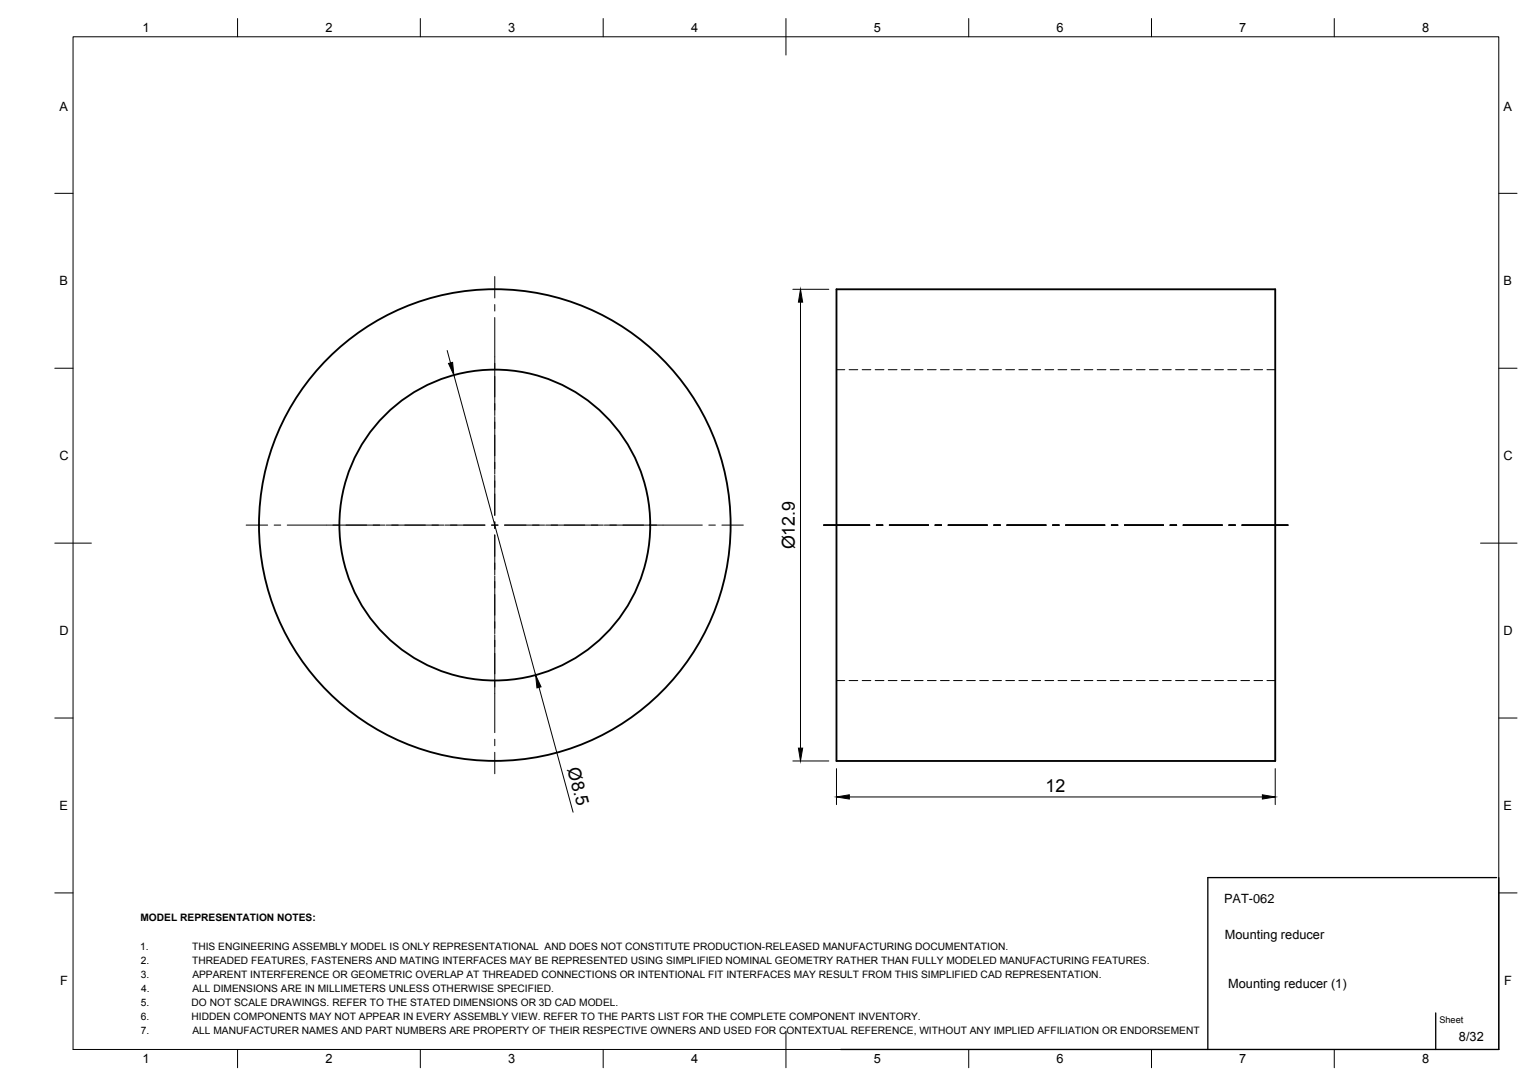
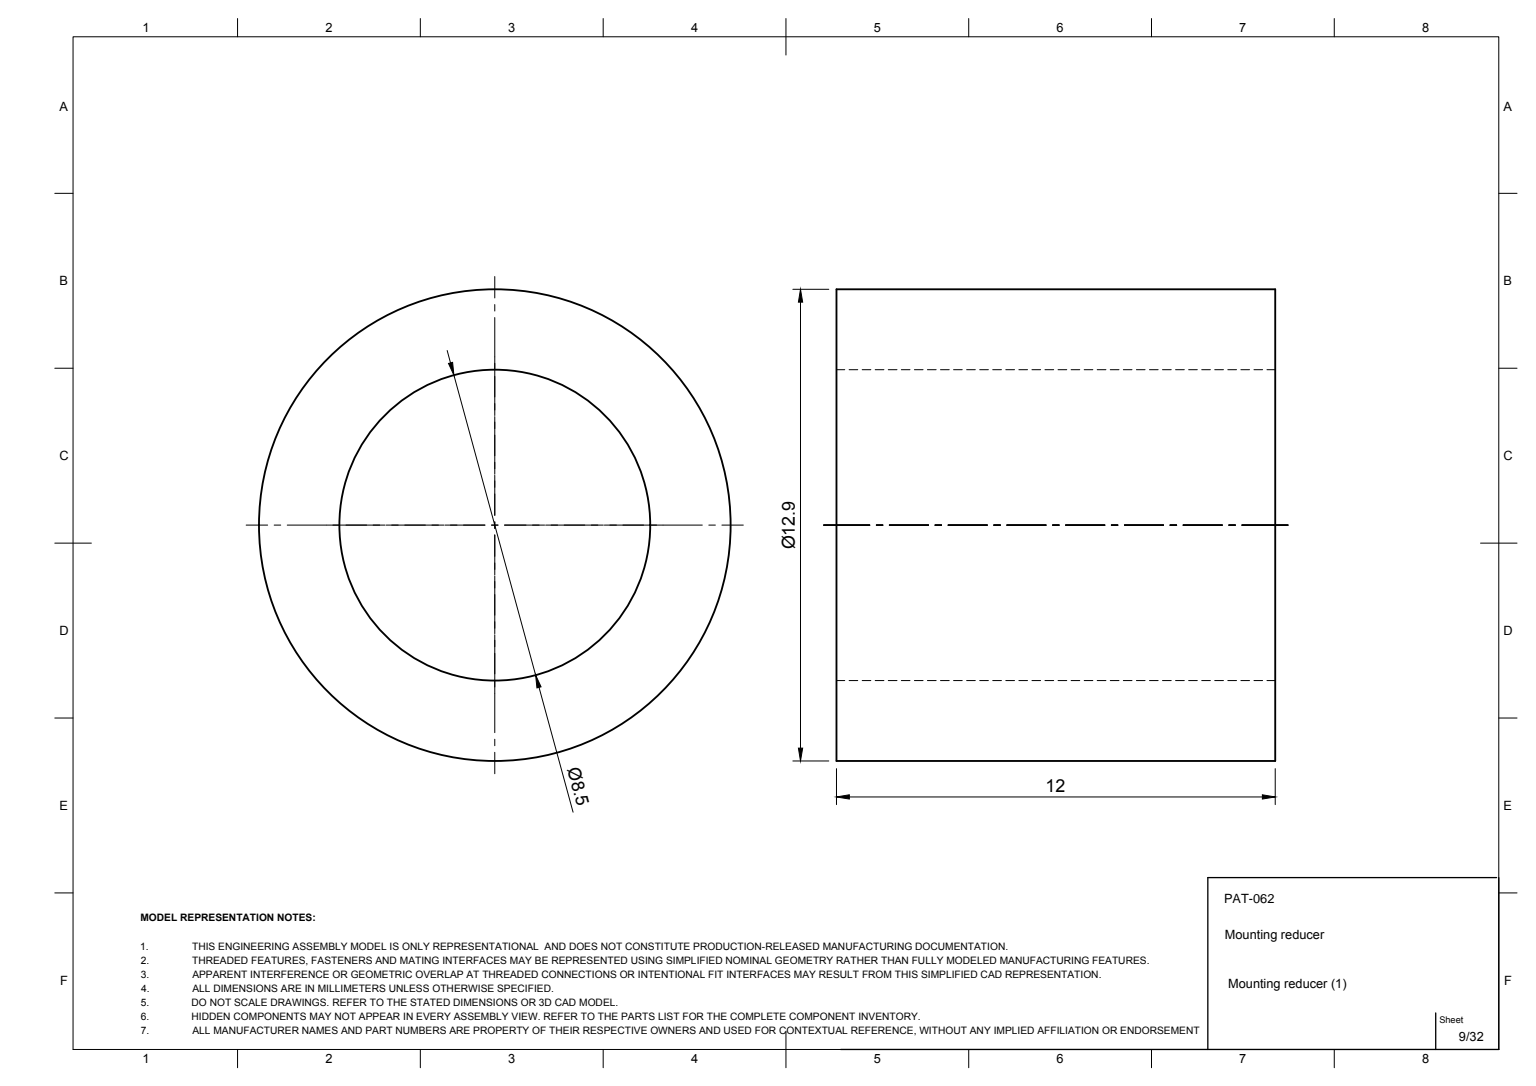
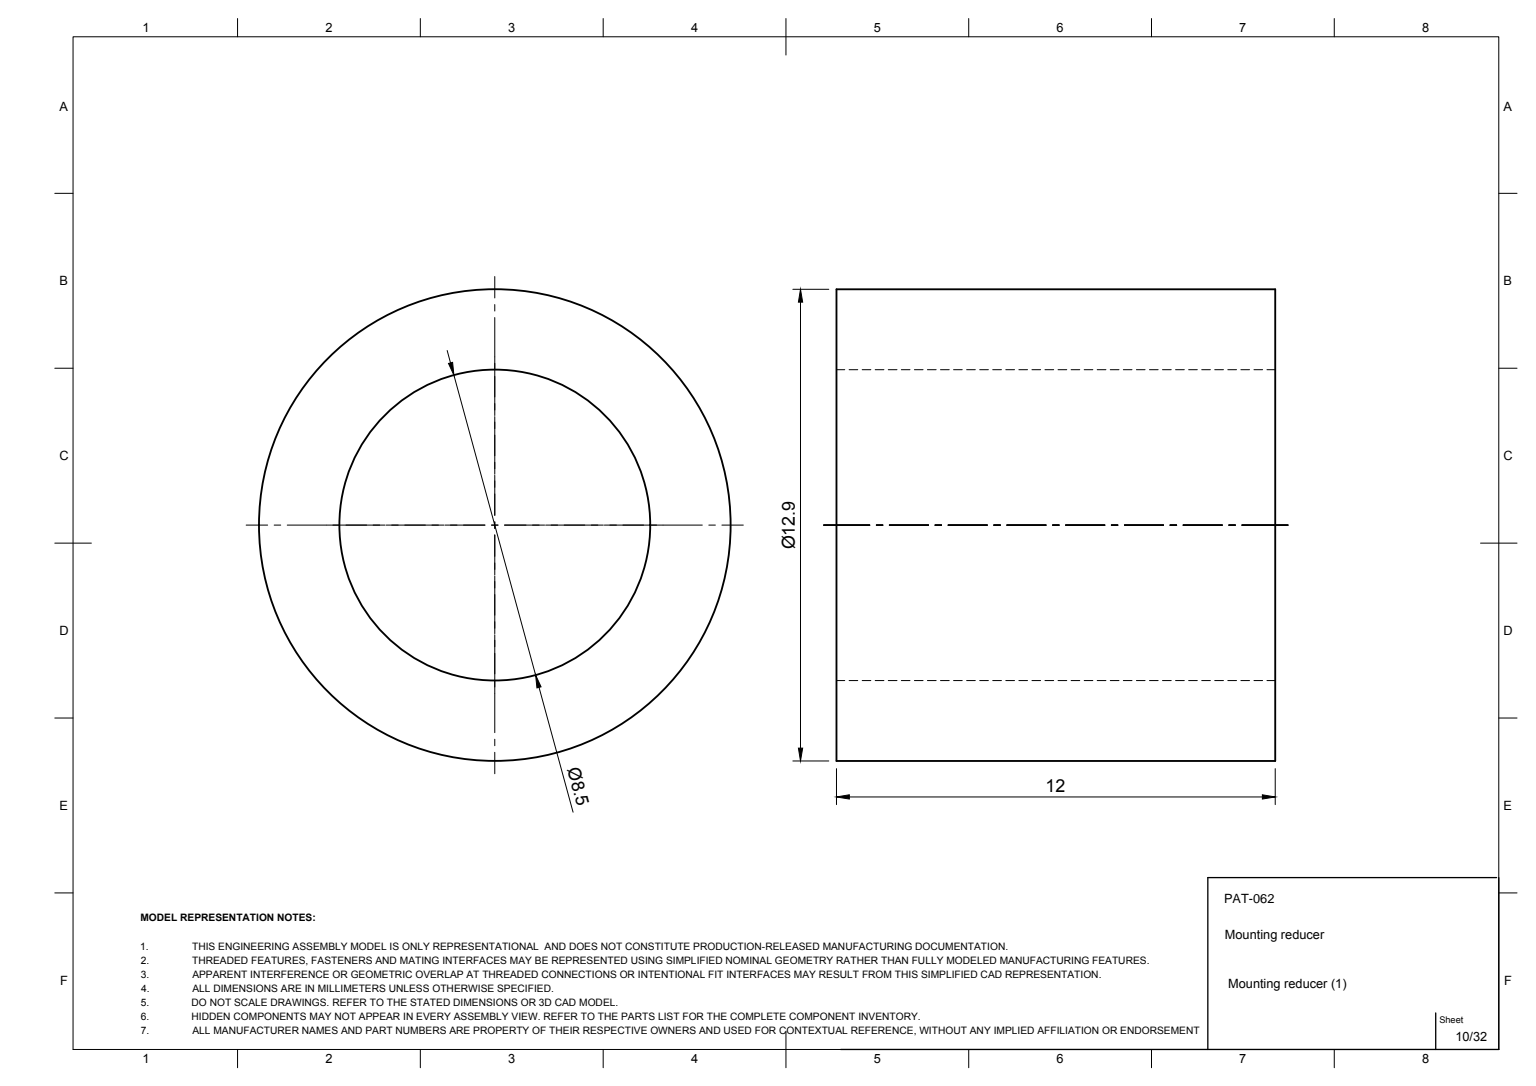
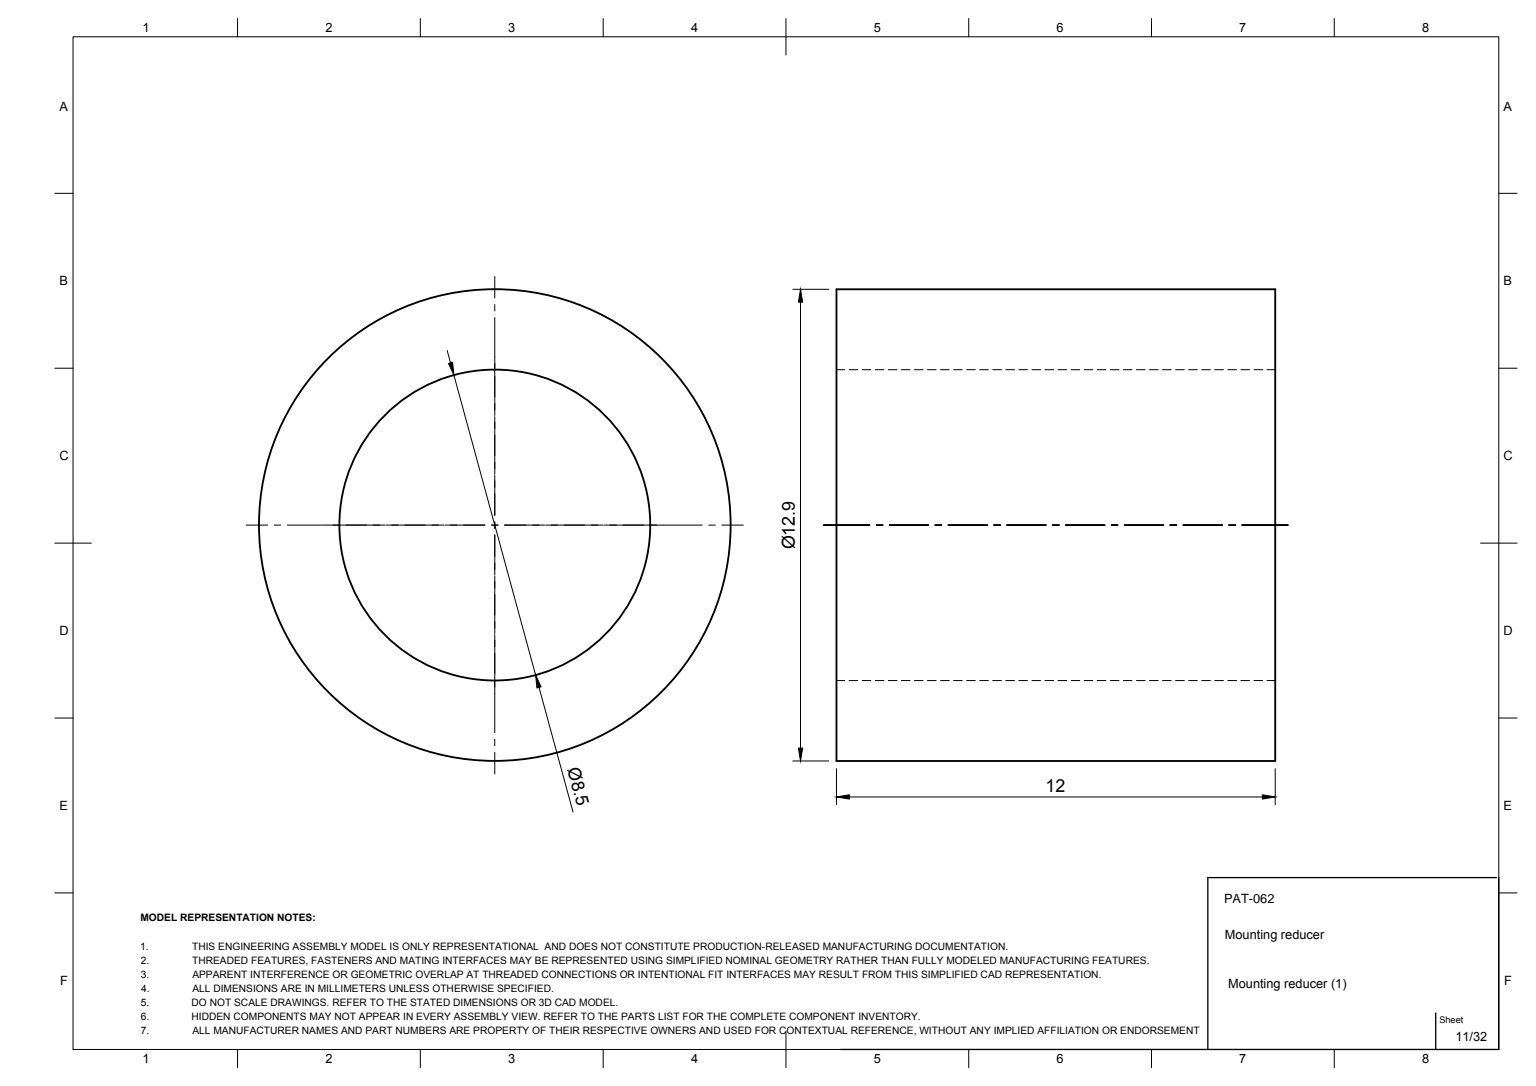
ISO-10303-21;
HEADER;
/* Generated by software containing ST-Developer
 * from STEP Tools, Inc. (www.steptools.com) 
 */

FILE_DESCRIPTION(
/* description */ ('Jaw-coupled motor to shaft test stand'),
/* implementation_level */ '2;1');

FILE_NAME(
/* name */ 'Mounting reducer.step',
/* time_stamp */ '2026-10-27T10:46:06-07:00',
/* author */ (''),
/* organization */ (''),
/* preprocessor_version */ 'ST-DEVELOPER v20.2',
/* originating_system */ 'Autodesk Translation Framework v15.17.0.0',
/* authorisation */ '');

FILE_SCHEMA (('AUTOMOTIVE_DESIGN { 1 0 10303 214 3 1 1 }'));
ENDSEC;

DATA;
#10=MECHANICAL_DESIGN_GEOMETRIC_PRESENTATION_REPRESENTATION('',(#343),#19361);
#279=SHAPE_REPRESENTATION_RELATIONSHIP('SRR','None',#19493,#311);
#311=ADVANCED_BREP_SHAPE_REPRESENTATION('',(#376),#19329);
#343=STYLED_ITEM('',(#19739),#376);
#376=MANIFOLD_SOLID_BREP('Body1',#10987);
#415=FACE_BOUND('',#1681,.T.);
#416=FACE_BOUND('',#1683,.T.);
#534=PLANE('',#11421);
#535=PLANE('',#11422);
#1046=FACE_OUTER_BOUND('',#1678,.T.);
#1047=FACE_OUTER_BOUND('',#1679,.T.);
#1048=FACE_OUTER_BOUND('',#1680,.T.);
#1049=FACE_OUTER_BOUND('',#1682,.T.);
#1678=EDGE_LOOP('',(#7454,#7455,#7456,#7457));
#1679=EDGE_LOOP('',(#7458,#7459,#7460,#7461));
#1680=EDGE_LOOP('',(#7462));
#1681=EDGE_LOOP('',(#7463));
#1682=EDGE_LOOP('',(#7464));
#1683=EDGE_LOOP('',(#7465));
#2417=LINE('',#15551,#3570);
#2418=LINE('',#15557,#3571);
#3570=VECTOR('',#12470,0.425);
#3571=VECTOR('',#12477,0.645);
#4693=CIRCLE('',#11416,0.425);
#4694=CIRCLE('',#11417,0.425);
#4695=CIRCLE('',#11419,0.645);
#4696=CIRCLE('',#11420,0.645);
#4979=VERTEX_POINT('',#15548);
#4980=VERTEX_POINT('',#15550);
#4981=VERTEX_POINT('',#15554);
#4982=VERTEX_POINT('',#15556);
#5938=EDGE_CURVE('',#4979,#4979,#4693,.T.);
#5939=EDGE_CURVE('',#4979,#4980,#2417,.T.);
#5940=EDGE_CURVE('',#4980,#4980,#4694,.T.);
#5941=EDGE_CURVE('',#4981,#4981,#4695,.T.);
#5942=EDGE_CURVE('',#4981,#4982,#2418,.T.);
#5943=EDGE_CURVE('',#4982,#4982,#4696,.T.);
#7454=ORIENTED_EDGE('',*,*,#5938,.F.);
#7455=ORIENTED_EDGE('',*,*,#5939,.T.);
#7456=ORIENTED_EDGE('',*,*,#5940,.T.);
#7457=ORIENTED_EDGE('',*,*,#5939,.F.);
#7458=ORIENTED_EDGE('',*,*,#5941,.F.);
#7459=ORIENTED_EDGE('',*,*,#5942,.T.);
#7460=ORIENTED_EDGE('',*,*,#5943,.T.);
#7461=ORIENTED_EDGE('',*,*,#5942,.F.);
#7462=ORIENTED_EDGE('',*,*,#5941,.T.);
#7463=ORIENTED_EDGE('',*,*,#5938,.T.);
#7464=ORIENTED_EDGE('',*,*,#5943,.F.);
#7465=ORIENTED_EDGE('',*,*,#5940,.F.);
#10276=CYLINDRICAL_SURFACE('',#11415,0.425);
#10277=CYLINDRICAL_SURFACE('',#11418,0.645);
#10388=ADVANCED_FACE('',(#1046),#10276,.F.);
#10389=ADVANCED_FACE('',(#1047),#10277,.T.);
#10390=ADVANCED_FACE('',(#1048,#415),#534,.T.);
#10391=ADVANCED_FACE('',(#1049,#416),#535,.F.);
#10987=CLOSED_SHELL('',(#10388,#10389,#10390,#10391));
#11414=AXIS2_PLACEMENT_3D('',#15546,#12464,#12465);
#11415=AXIS2_PLACEMENT_3D('',#15547,#12466,#12467);
#11416=AXIS2_PLACEMENT_3D('',#15549,#12468,#12469);
#11417=AXIS2_PLACEMENT_3D('',#15552,#12471,#12472);
#11418=AXIS2_PLACEMENT_3D('',#15553,#12473,#12474);
#11419=AXIS2_PLACEMENT_3D('',#15555,#12475,#12476);
#11420=AXIS2_PLACEMENT_3D('',#15558,#12478,#12479);
#11421=AXIS2_PLACEMENT_3D('',#15559,#12480,#12481);
#11422=AXIS2_PLACEMENT_3D('',#15560,#12482,#12483);
#12464=DIRECTION('axis',(0.,0.,1.));
#12465=DIRECTION('refdir',(1.,0.,0.));
#12466=DIRECTION('center_axis',(0.,0.,1.));
#12467=DIRECTION('ref_axis',(1.,0.,0.));
#12468=DIRECTION('center_axis',(0.,0.,-1.));
#12469=DIRECTION('ref_axis',(1.,0.,0.));
#12470=DIRECTION('',(0.,0.,-1.));
#12471=DIRECTION('center_axis',(0.,0.,-1.));
#12472=DIRECTION('ref_axis',(1.,0.,0.));
#12473=DIRECTION('center_axis',(0.,0.,1.));
#12474=DIRECTION('ref_axis',(1.,0.,0.));
#12475=DIRECTION('center_axis',(0.,0.,1.));
#12476=DIRECTION('ref_axis',(1.,0.,0.));
#12477=DIRECTION('',(0.,0.,-1.));
#12478=DIRECTION('center_axis',(0.,0.,1.));
#12479=DIRECTION('ref_axis',(1.,0.,0.));
#12480=DIRECTION('center_axis',(0.,0.,1.));
#12481=DIRECTION('ref_axis',(1.,0.,0.));
#12482=DIRECTION('center_axis',(0.,0.,1.));
#12483=DIRECTION('ref_axis',(1.,0.,0.));
#15546=CARTESIAN_POINT('',(0.,0.,0.));
#15547=CARTESIAN_POINT('Origin',(-4.75,2.,1.2));
#15548=CARTESIAN_POINT('',(-5.175,2.,2.4));
#15549=CARTESIAN_POINT('Origin',(-4.75,2.,2.4));
#15550=CARTESIAN_POINT('',(-5.175,2.,1.2));
#15551=CARTESIAN_POINT('',(-5.175,2.,1.2));
#15552=CARTESIAN_POINT('Origin',(-4.75,2.,1.2));
#15553=CARTESIAN_POINT('Origin',(-4.75,2.,1.2));
#15554=CARTESIAN_POINT('',(-5.395,2.,2.4));
#15555=CARTESIAN_POINT('Origin',(-4.75,2.,2.4));
#15556=CARTESIAN_POINT('',(-5.395,2.,1.2));
#15557=CARTESIAN_POINT('',(-5.395,2.,1.2));
#15558=CARTESIAN_POINT('Origin',(-4.75,2.,1.2));
#15559=CARTESIAN_POINT('Origin',(-4.75,2.,2.4));
#15560=CARTESIAN_POINT('Origin',(-4.75,2.,1.2));
#19291=UNCERTAINTY_MEASURE_WITH_UNIT(LENGTH_MEASURE(0.001),#19362,
'DISTANCE_ACCURACY_VALUE',
'Maximum model space distance between geometric entities at asserted c
onnectivities');
#19323=UNCERTAINTY_MEASURE_WITH_UNIT(LENGTH_MEASURE(0.001),#19362,
'DISTANCE_ACCURACY_VALUE',
'Maximum model space distance between geometric entities at asserted c
onnectivities');
#19329=(
GEOMETRIC_REPRESENTATION_CONTEXT(3)
GLOBAL_UNCERTAINTY_ASSIGNED_CONTEXT((#19291))
GLOBAL_UNIT_ASSIGNED_CONTEXT((#19362,#19364,#19365))
REPRESENTATION_CONTEXT('','3D')
);
#19361=(
GEOMETRIC_REPRESENTATION_CONTEXT(3)
GLOBAL_UNCERTAINTY_ASSIGNED_CONTEXT((#19323))
GLOBAL_UNIT_ASSIGNED_CONTEXT((#19362,#19364,#19365))
REPRESENTATION_CONTEXT('','3D')
);
#19362=(
LENGTH_UNIT()
NAMED_UNIT(*)
SI_UNIT(.CENTI.,.METRE.)
);
#19364=(
NAMED_UNIT(*)
PLANE_ANGLE_UNIT()
SI_UNIT($,.RADIAN.)
);
#19365=(
NAMED_UNIT(*)
SI_UNIT($,.STERADIAN.)
SOLID_ANGLE_UNIT()
);
#19371=SHAPE_DEFINITION_REPRESENTATION(#19408,#19493);
#19408=PRODUCT_DEFINITION_SHAPE('',$,#19531);
#19493=SHAPE_REPRESENTATION('',(#11414),#19329);
#19525=PRODUCT_DEFINITION_CONTEXT('part definition',#19638,'design');
#19531=PRODUCT_DEFINITION('Mounting reducer','Mounting reducer',#19568,
#19525);
#19568=PRODUCT_DEFINITION_FORMATION('',$,#19645);
#19638=APPLICATION_CONTEXT(
'Core Data for Automotive Mechanical Design Process');
#19639=PRODUCT_CONTEXT('part definition',#19638,'mechanical');
#19645=PRODUCT('Mounting reducer','Mounting reducer','Mounting reducer',
(#19639));
#19733=COLOUR_RGB('Sky Blue',0.24,0.69,0.87);
#19734=FILL_AREA_STYLE_COLOUR('',#19733);
#19735=FILL_AREA_STYLE('',(#19734));
#19736=SURFACE_STYLE_FILL_AREA(#19735);
#19737=SURFACE_SIDE_STYLE('',(#19736));
#19738=SURFACE_STYLE_USAGE(.BOTH.,#19737);
#19739=PRESENTATION_STYLE_ASSIGNMENT((#19738));
ENDSEC;
END-ISO-10303-21;
